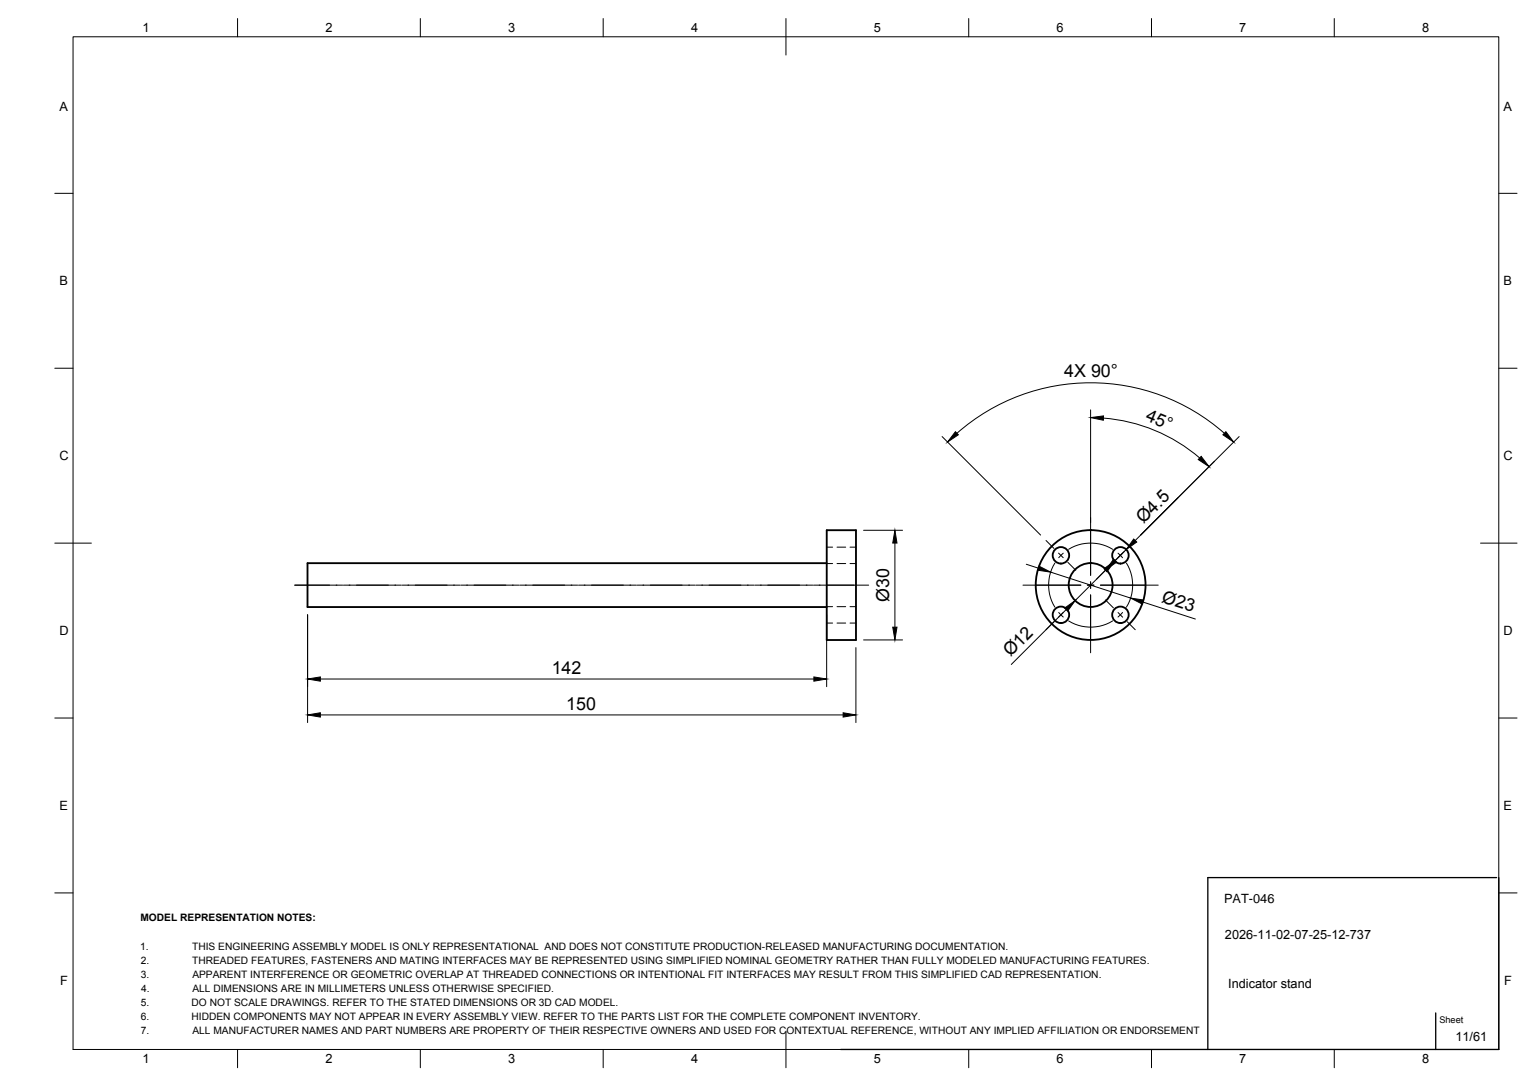
ISO-10303-21;
HEADER;
/* Generated by software containing ST-Developer
 * from STEP Tools, Inc. (www.steptools.com) 
 */

FILE_DESCRIPTION(
/* description */ ('Gear mesh backlash fixture'),
/* implementation_level */ '2;1');

FILE_NAME(
/* name */ 'Indicator stand.step',
/* time_stamp */ '2026-10-28T03:26:00-07:00',
/* author */ (''),
/* organization */ (''),
/* preprocessor_version */ 'ST-DEVELOPER v20.2',
/* originating_system */ 'Autodesk Translation Framework v15.17.0.0',
/* authorisation */ '');

FILE_SCHEMA (('AUTOMOTIVE_DESIGN { 1 0 10303 214 3 1 1 }'));
ENDSEC;

DATA;
#10=MECHANICAL_DESIGN_GEOMETRIC_PRESENTATION_REPRESENTATION('',(#1022),#57900);
#922=SHAPE_REPRESENTATION_RELATIONSHIP('SRR','None',#58117,#972);
#972=ADVANCED_BREP_SHAPE_REPRESENTATION('',(#1087),#57850);
#1022=STYLED_ITEM('',(#58458),#1087);
#1087=MANIFOLD_SOLID_BREP('Body1',#13582);
#1190=FACE_BOUND('',#2590,.T.);
#1191=FACE_BOUND('',#2591,.T.);
#1192=FACE_BOUND('',#2592,.T.);
#1193=FACE_BOUND('',#2593,.T.);
#1194=FACE_BOUND('',#2594,.T.);
#1195=FACE_BOUND('',#2596,.T.);
#1196=FACE_BOUND('',#2597,.T.);
#1197=FACE_BOUND('',#2598,.T.);
#1198=FACE_BOUND('',#2599,.T.);
#1365=PLANE('',#14383);
#1366=PLANE('',#14387);
#1367=PLANE('',#14388);
#1770=FACE_OUTER_BOUND('',#2582,.T.);
#1771=FACE_OUTER_BOUND('',#2583,.T.);
#1772=FACE_OUTER_BOUND('',#2584,.T.);
#1773=FACE_OUTER_BOUND('',#2585,.T.);
#1774=FACE_OUTER_BOUND('',#2586,.T.);
#1775=FACE_OUTER_BOUND('',#2587,.T.);
#1776=FACE_OUTER_BOUND('',#2588,.T.);
#1777=FACE_OUTER_BOUND('',#2589,.T.);
#1778=FACE_OUTER_BOUND('',#2595,.T.);
#2582=EDGE_LOOP('',(#9225,#9226,#9227,#9228));
#2583=EDGE_LOOP('',(#9229,#9230,#9231,#9232));
#2584=EDGE_LOOP('',(#9233,#9234,#9235,#9236));
#2585=EDGE_LOOP('',(#9237,#9238,#9239,#9240));
#2586=EDGE_LOOP('',(#9241,#9242,#9243,#9244));
#2587=EDGE_LOOP('',(#9245));
#2588=EDGE_LOOP('',(#9246,#9247,#9248,#9249));
#2589=EDGE_LOOP('',(#9250));
#2590=EDGE_LOOP('',(#9251));
#2591=EDGE_LOOP('',(#9252));
#2592=EDGE_LOOP('',(#9253));
#2593=EDGE_LOOP('',(#9254));
#2594=EDGE_LOOP('',(#9255));
#2595=EDGE_LOOP('',(#9256));
#2596=EDGE_LOOP('',(#9257));
#2597=EDGE_LOOP('',(#9258));
#2598=EDGE_LOOP('',(#9259));
#2599=EDGE_LOOP('',(#9260));
#3492=LINE('',#19679,#4381);
#3493=LINE('',#19685,#4382);
#3494=LINE('',#19691,#4383);
#3495=LINE('',#19697,#4384);
#3496=LINE('',#19703,#4385);
#3497=LINE('',#19710,#4386);
#4381=VECTOR('',#16009,0.225);
#4382=VECTOR('',#16016,0.225);
#4383=VECTOR('',#16023,0.225);
#4384=VECTOR('',#16030,0.225);
#4385=VECTOR('',#16037,0.6);
#4386=VECTOR('',#16046,1.5);
#5277=CIRCLE('',#14369,0.225);
#5278=CIRCLE('',#14370,0.225);
#5279=CIRCLE('',#14372,0.225);
#5280=CIRCLE('',#14373,0.225);
#5281=CIRCLE('',#14375,0.225);
#5282=CIRCLE('',#14376,0.225);
#5283=CIRCLE('',#14378,0.225);
#5284=CIRCLE('',#14379,0.225);
#5285=CIRCLE('',#14381,0.6);
#5286=CIRCLE('',#14382,0.6);
#5287=CIRCLE('',#14385,1.5);
#5288=CIRCLE('',#14386,1.5);
#5897=VERTEX_POINT('',#19676);
#5898=VERTEX_POINT('',#19678);
#5899=VERTEX_POINT('',#19682);
#5900=VERTEX_POINT('',#19684);
#5901=VERTEX_POINT('',#19688);
#5902=VERTEX_POINT('',#19690);
#5903=VERTEX_POINT('',#19694);
#5904=VERTEX_POINT('',#19696);
#5905=VERTEX_POINT('',#19700);
#5906=VERTEX_POINT('',#19702);
#5907=VERTEX_POINT('',#19707);
#5908=VERTEX_POINT('',#19709);
#7199=EDGE_CURVE('',#5897,#5897,#5277,.T.);
#7200=EDGE_CURVE('',#5897,#5898,#3492,.T.);
#7201=EDGE_CURVE('',#5898,#5898,#5278,.T.);
#7202=EDGE_CURVE('',#5899,#5899,#5279,.T.);
#7203=EDGE_CURVE('',#5899,#5900,#3493,.T.);
#7204=EDGE_CURVE('',#5900,#5900,#5280,.T.);
#7205=EDGE_CURVE('',#5901,#5901,#5281,.T.);
#7206=EDGE_CURVE('',#5901,#5902,#3494,.T.);
#7207=EDGE_CURVE('',#5902,#5902,#5282,.T.);
#7208=EDGE_CURVE('',#5903,#5903,#5283,.T.);
#7209=EDGE_CURVE('',#5903,#5904,#3495,.T.);
#7210=EDGE_CURVE('',#5904,#5904,#5284,.T.);
#7211=EDGE_CURVE('',#5905,#5905,#5285,.T.);
#7212=EDGE_CURVE('',#5905,#5906,#3496,.T.);
#7213=EDGE_CURVE('',#5906,#5906,#5286,.T.);
#7214=EDGE_CURVE('',#5907,#5907,#5287,.T.);
#7215=EDGE_CURVE('',#5907,#5908,#3497,.T.);
#7216=EDGE_CURVE('',#5908,#5908,#5288,.T.);
#9225=ORIENTED_EDGE('',*,*,#7199,.F.);
#9226=ORIENTED_EDGE('',*,*,#7200,.T.);
#9227=ORIENTED_EDGE('',*,*,#7201,.F.);
#9228=ORIENTED_EDGE('',*,*,#7200,.F.);
#9229=ORIENTED_EDGE('',*,*,#7202,.F.);
#9230=ORIENTED_EDGE('',*,*,#7203,.T.);
#9231=ORIENTED_EDGE('',*,*,#7204,.F.);
#9232=ORIENTED_EDGE('',*,*,#7203,.F.);
#9233=ORIENTED_EDGE('',*,*,#7205,.F.);
#9234=ORIENTED_EDGE('',*,*,#7206,.T.);
#9235=ORIENTED_EDGE('',*,*,#7207,.F.);
#9236=ORIENTED_EDGE('',*,*,#7206,.F.);
#9237=ORIENTED_EDGE('',*,*,#7208,.F.);
#9238=ORIENTED_EDGE('',*,*,#7209,.T.);
#9239=ORIENTED_EDGE('',*,*,#7210,.F.);
#9240=ORIENTED_EDGE('',*,*,#7209,.F.);
#9241=ORIENTED_EDGE('',*,*,#7211,.F.);
#9242=ORIENTED_EDGE('',*,*,#7212,.T.);
#9243=ORIENTED_EDGE('',*,*,#7213,.F.);
#9244=ORIENTED_EDGE('',*,*,#7212,.F.);
#9245=ORIENTED_EDGE('',*,*,#7211,.T.);
#9246=ORIENTED_EDGE('',*,*,#7214,.F.);
#9247=ORIENTED_EDGE('',*,*,#7215,.T.);
#9248=ORIENTED_EDGE('',*,*,#7216,.T.);
#9249=ORIENTED_EDGE('',*,*,#7215,.F.);
#9250=ORIENTED_EDGE('',*,*,#7214,.T.);
#9251=ORIENTED_EDGE('',*,*,#7213,.T.);
#9252=ORIENTED_EDGE('',*,*,#7210,.T.);
#9253=ORIENTED_EDGE('',*,*,#7207,.T.);
#9254=ORIENTED_EDGE('',*,*,#7204,.T.);
#9255=ORIENTED_EDGE('',*,*,#7201,.T.);
#9256=ORIENTED_EDGE('',*,*,#7216,.F.);
#9257=ORIENTED_EDGE('',*,*,#7199,.T.);
#9258=ORIENTED_EDGE('',*,*,#7202,.T.);
#9259=ORIENTED_EDGE('',*,*,#7205,.T.);
#9260=ORIENTED_EDGE('',*,*,#7208,.T.);
#12626=CYLINDRICAL_SURFACE('',#14368,0.225);
#12627=CYLINDRICAL_SURFACE('',#14371,0.225);
#12628=CYLINDRICAL_SURFACE('',#14374,0.225);
#12629=CYLINDRICAL_SURFACE('',#14377,0.225);
#12630=CYLINDRICAL_SURFACE('',#14380,0.6);
#12631=CYLINDRICAL_SURFACE('',#14384,1.5);
#12887=ADVANCED_FACE('',(#1770),#12626,.F.);
#12888=ADVANCED_FACE('',(#1771),#12627,.F.);
#12889=ADVANCED_FACE('',(#1772),#12628,.F.);
#12890=ADVANCED_FACE('',(#1773),#12629,.F.);
#12891=ADVANCED_FACE('',(#1774),#12630,.T.);
#12892=ADVANCED_FACE('',(#1775),#1365,.T.);
#12893=ADVANCED_FACE('',(#1776),#12631,.T.);
#12894=ADVANCED_FACE('',(#1777,#1190,#1191,#1192,#1193,#1194),#1366,.T.);
#12895=ADVANCED_FACE('',(#1778,#1195,#1196,#1197,#1198),#1367,.F.);
#13582=CLOSED_SHELL('',(#12887,#12888,#12889,#12890,#12891,#12892,#12893,
#12894,#12895));
#14367=AXIS2_PLACEMENT_3D('',#19674,#16003,#16004);
#14368=AXIS2_PLACEMENT_3D('',#19675,#16005,#16006);
#14369=AXIS2_PLACEMENT_3D('',#19677,#16007,#16008);
#14370=AXIS2_PLACEMENT_3D('',#19680,#16010,#16011);
#14371=AXIS2_PLACEMENT_3D('',#19681,#16012,#16013);
#14372=AXIS2_PLACEMENT_3D('',#19683,#16014,#16015);
#14373=AXIS2_PLACEMENT_3D('',#19686,#16017,#16018);
#14374=AXIS2_PLACEMENT_3D('',#19687,#16019,#16020);
#14375=AXIS2_PLACEMENT_3D('',#19689,#16021,#16022);
#14376=AXIS2_PLACEMENT_3D('',#19692,#16024,#16025);
#14377=AXIS2_PLACEMENT_3D('',#19693,#16026,#16027);
#14378=AXIS2_PLACEMENT_3D('',#19695,#16028,#16029);
#14379=AXIS2_PLACEMENT_3D('',#19698,#16031,#16032);
#14380=AXIS2_PLACEMENT_3D('',#19699,#16033,#16034);
#14381=AXIS2_PLACEMENT_3D('',#19701,#16035,#16036);
#14382=AXIS2_PLACEMENT_3D('',#19704,#16038,#16039);
#14383=AXIS2_PLACEMENT_3D('',#19705,#16040,#16041);
#14384=AXIS2_PLACEMENT_3D('',#19706,#16042,#16043);
#14385=AXIS2_PLACEMENT_3D('',#19708,#16044,#16045);
#14386=AXIS2_PLACEMENT_3D('',#19711,#16047,#16048);
#14387=AXIS2_PLACEMENT_3D('',#19712,#16049,#16050);
#14388=AXIS2_PLACEMENT_3D('',#19713,#16051,#16052);
#16003=DIRECTION('axis',(0.,0.,1.));
#16004=DIRECTION('refdir',(1.,0.,0.));
#16005=DIRECTION('center_axis',(0.,0.,1.));
#16006=DIRECTION('ref_axis',(1.,0.,0.));
#16007=DIRECTION('center_axis',(0.,0.,1.));
#16008=DIRECTION('ref_axis',(1.,0.,0.));
#16009=DIRECTION('',(0.,0.,1.));
#16010=DIRECTION('center_axis',(0.,0.,-1.));
#16011=DIRECTION('ref_axis',(1.,0.,0.));
#16012=DIRECTION('center_axis',(0.,0.,1.));
#16013=DIRECTION('ref_axis',(1.,0.,0.));
#16014=DIRECTION('center_axis',(0.,0.,1.));
#16015=DIRECTION('ref_axis',(1.,0.,0.));
#16016=DIRECTION('',(0.,0.,1.));
#16017=DIRECTION('center_axis',(0.,0.,-1.));
#16018=DIRECTION('ref_axis',(1.,0.,0.));
#16019=DIRECTION('center_axis',(0.,0.,1.));
#16020=DIRECTION('ref_axis',(1.,0.,0.));
#16021=DIRECTION('center_axis',(0.,0.,1.));
#16022=DIRECTION('ref_axis',(1.,0.,0.));
#16023=DIRECTION('',(0.,0.,1.));
#16024=DIRECTION('center_axis',(0.,0.,-1.));
#16025=DIRECTION('ref_axis',(1.,0.,0.));
#16026=DIRECTION('center_axis',(0.,0.,1.));
#16027=DIRECTION('ref_axis',(1.,0.,0.));
#16028=DIRECTION('center_axis',(0.,0.,1.));
#16029=DIRECTION('ref_axis',(1.,0.,0.));
#16030=DIRECTION('',(0.,0.,1.));
#16031=DIRECTION('center_axis',(0.,0.,-1.));
#16032=DIRECTION('ref_axis',(1.,0.,0.));
#16033=DIRECTION('center_axis',(0.,0.,1.));
#16034=DIRECTION('ref_axis',(1.,0.,0.));
#16035=DIRECTION('center_axis',(0.,0.,1.));
#16036=DIRECTION('ref_axis',(1.,0.,0.));
#16037=DIRECTION('',(0.,0.,-1.));
#16038=DIRECTION('center_axis',(0.,0.,-1.));
#16039=DIRECTION('ref_axis',(1.,0.,0.));
#16040=DIRECTION('center_axis',(0.,0.,1.));
#16041=DIRECTION('ref_axis',(1.,0.,0.));
#16042=DIRECTION('center_axis',(0.,0.,1.));
#16043=DIRECTION('ref_axis',(1.,0.,0.));
#16044=DIRECTION('center_axis',(0.,0.,1.));
#16045=DIRECTION('ref_axis',(1.,0.,0.));
#16046=DIRECTION('',(0.,0.,-1.));
#16047=DIRECTION('center_axis',(0.,0.,1.));
#16048=DIRECTION('ref_axis',(1.,0.,0.));
#16049=DIRECTION('center_axis',(0.,0.,1.));
#16050=DIRECTION('ref_axis',(1.,0.,0.));
#16051=DIRECTION('center_axis',(0.,0.,1.));
#16052=DIRECTION('ref_axis',(1.,0.,0.));
#19674=CARTESIAN_POINT('',(0.,0.,0.));
#19675=CARTESIAN_POINT('Origin',(11.1868272016355,8.18682720163547,-0.1));
#19676=CARTESIAN_POINT('',(10.9618272016355,8.18682720163547,0.));
#19677=CARTESIAN_POINT('Origin',(11.1868272016355,8.18682720163547,0.));
#19678=CARTESIAN_POINT('',(10.9618272016355,8.18682720163547,0.8));
#19679=CARTESIAN_POINT('',(10.9618272016355,8.18682720163547,-0.1));
#19680=CARTESIAN_POINT('Origin',(11.1868272016355,8.18682720163547,0.8));
#19681=CARTESIAN_POINT('Origin',(11.1868272016355,9.81317279836453,-0.1));
#19682=CARTESIAN_POINT('',(10.9618272016355,9.81317279836453,0.));
#19683=CARTESIAN_POINT('Origin',(11.1868272016355,9.81317279836453,0.));
#19684=CARTESIAN_POINT('',(10.9618272016355,9.81317279836453,0.8));
#19685=CARTESIAN_POINT('',(10.9618272016355,9.81317279836453,-0.1));
#19686=CARTESIAN_POINT('Origin',(11.1868272016355,9.81317279836453,0.8));
#19687=CARTESIAN_POINT('Origin',(12.8131727983645,9.81317279836453,-0.1));
#19688=CARTESIAN_POINT('',(12.5881727983645,9.81317279836453,0.));
#19689=CARTESIAN_POINT('Origin',(12.8131727983645,9.81317279836453,0.));
#19690=CARTESIAN_POINT('',(12.5881727983645,9.81317279836453,0.8));
#19691=CARTESIAN_POINT('',(12.5881727983645,9.81317279836453,-0.1));
#19692=CARTESIAN_POINT('Origin',(12.8131727983645,9.81317279836453,0.8));
#19693=CARTESIAN_POINT('Origin',(12.8131727983645,8.18682720163547,-0.1));
#19694=CARTESIAN_POINT('',(12.5881727983645,8.18682720163547,0.));
#19695=CARTESIAN_POINT('Origin',(12.8131727983645,8.18682720163547,0.));
#19696=CARTESIAN_POINT('',(12.5881727983645,8.18682720163547,0.8));
#19697=CARTESIAN_POINT('',(12.5881727983645,8.18682720163547,-0.1));
#19698=CARTESIAN_POINT('Origin',(12.8131727983645,8.18682720163547,0.8));
#19699=CARTESIAN_POINT('Origin',(12.,9.,0.8));
#19700=CARTESIAN_POINT('',(11.4,9.,15.));
#19701=CARTESIAN_POINT('Origin',(12.,9.,15.));
#19702=CARTESIAN_POINT('',(11.4,9.,0.8));
#19703=CARTESIAN_POINT('',(11.4,9.,0.8));
#19704=CARTESIAN_POINT('Origin',(12.,9.,0.8));
#19705=CARTESIAN_POINT('Origin',(12.,9.,15.));
#19706=CARTESIAN_POINT('Origin',(12.,9.,0.));
#19707=CARTESIAN_POINT('',(10.5,9.,0.8));
#19708=CARTESIAN_POINT('Origin',(12.,9.,0.8));
#19709=CARTESIAN_POINT('',(10.5,9.,0.));
#19710=CARTESIAN_POINT('',(10.5,9.,0.));
#19711=CARTESIAN_POINT('Origin',(12.,9.,0.));
#19712=CARTESIAN_POINT('Origin',(12.,9.,0.8));
#19713=CARTESIAN_POINT('Origin',(12.,9.,0.));
#57791=UNCERTAINTY_MEASURE_WITH_UNIT(LENGTH_MEASURE(0.001),#57901,
'DISTANCE_ACCURACY_VALUE',
'Maximum model space distance between geometric entities at asserted c
onnectivities');
#57841=UNCERTAINTY_MEASURE_WITH_UNIT(LENGTH_MEASURE(0.001),#57901,
'DISTANCE_ACCURACY_VALUE',
'Maximum model space distance between geometric entities at asserted c
onnectivities');
#57850=(
GEOMETRIC_REPRESENTATION_CONTEXT(3)
GLOBAL_UNCERTAINTY_ASSIGNED_CONTEXT((#57791))
GLOBAL_UNIT_ASSIGNED_CONTEXT((#57901,#57903,#57904))
REPRESENTATION_CONTEXT('','3D')
);
#57900=(
GEOMETRIC_REPRESENTATION_CONTEXT(3)
GLOBAL_UNCERTAINTY_ASSIGNED_CONTEXT((#57841))
GLOBAL_UNIT_ASSIGNED_CONTEXT((#57901,#57903,#57904))
REPRESENTATION_CONTEXT('','3D')
);
#57901=(
LENGTH_UNIT()
NAMED_UNIT(*)
SI_UNIT(.CENTI.,.METRE.)
);
#57903=(
NAMED_UNIT(*)
PLANE_ANGLE_UNIT()
SI_UNIT($,.RADIAN.)
);
#57904=(
NAMED_UNIT(*)
SI_UNIT($,.STERADIAN.)
SOLID_ANGLE_UNIT()
);
#57913=SHAPE_DEFINITION_REPRESENTATION(#57971,#58117);
#57971=PRODUCT_DEFINITION_SHAPE('',$,#58176);
#58117=SHAPE_REPRESENTATION('',(#14367),#57850);
#58167=PRODUCT_DEFINITION_CONTEXT('part definition',#58343,'design');
#58176=PRODUCT_DEFINITION('Indicator stand','Indicator stand',#58234,#58167);
#58234=PRODUCT_DEFINITION_FORMATION('',$,#58353);
#58343=APPLICATION_CONTEXT(
'Core Data for Automotive Mechanical Design Process');
#58344=PRODUCT_CONTEXT('part definition',#58343,'mechanical');
#58353=PRODUCT('Indicator stand','Indicator stand','Indicator stand',(#58344));
#58452=COLOUR_RGB('Sky Blue',0.24,0.69,0.87);
#58453=FILL_AREA_STYLE_COLOUR('',#58452);
#58454=FILL_AREA_STYLE('',(#58453));
#58455=SURFACE_STYLE_FILL_AREA(#58454);
#58456=SURFACE_SIDE_STYLE('',(#58455));
#58457=SURFACE_STYLE_USAGE(.BOTH.,#58456);
#58458=PRESENTATION_STYLE_ASSIGNMENT((#58457));
ENDSEC;
END-ISO-10303-21;
